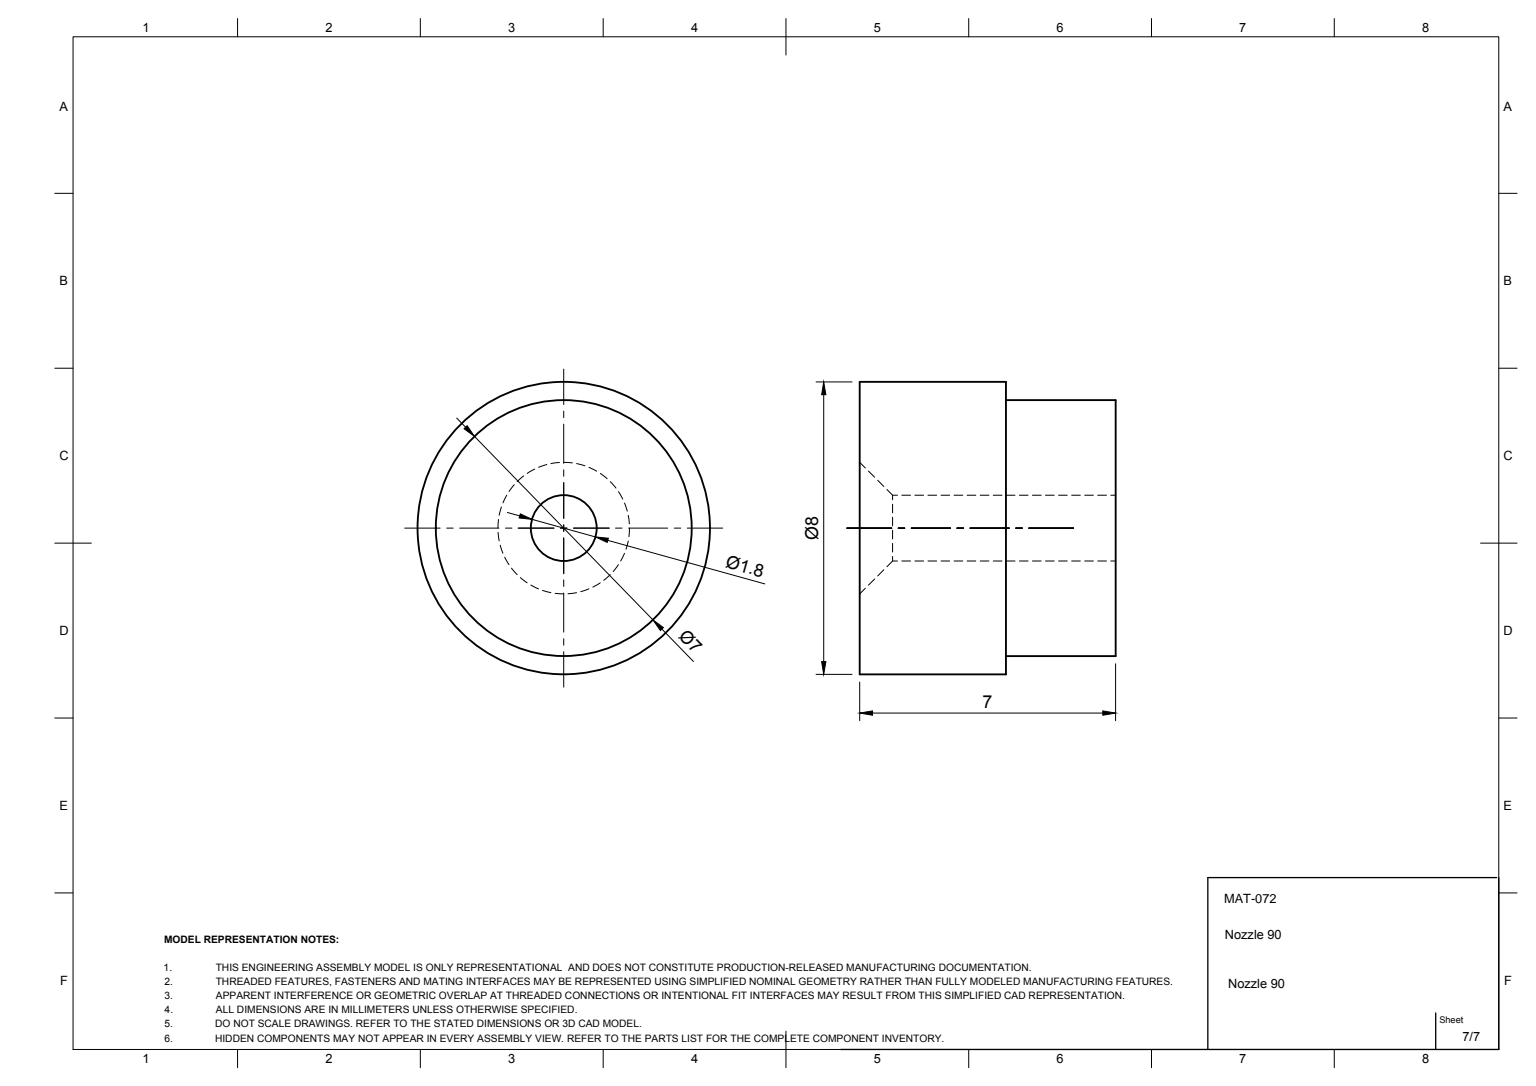
ISO-10303-21;
HEADER;
/* Generated by software containing ST-Developer
 * from STEP Tools, Inc. (www.steptools.com) 
 */

FILE_DESCRIPTION(
/* description */ (''),
/* implementation_level */ '2;1');

FILE_NAME(
/* name */ 'Nozzle 90.step',
/* time_stamp */ '2026-10-24T10:30:45-07:00',
/* author */ (''),
/* organization */ (''),
/* preprocessor_version */ 'ST-DEVELOPER v20.2',
/* originating_system */ 'Autodesk Translation Framework v15.15.0.0',
/* authorisation */ '');

FILE_SCHEMA (('AUTOMOTIVE_DESIGN { 1 0 10303 214 3 1 1 }'));
ENDSEC;

DATA;
#10=MECHANICAL_DESIGN_GEOMETRIC_PRESENTATION_REPRESENTATION('',(#81),#5183);
#66=CONICAL_SURFACE('',#2661,1.8,0.785398163397448);
#71=SHAPE_REPRESENTATION_RELATIONSHIP('SRR','None',#5218,#76);
#76=ADVANCED_BREP_SHAPE_REPRESENTATION('',(#86),#5182);
#81=STYLED_ITEM('',(#5247),#86);
#86=MANIFOLD_SOLID_BREP('Nozzle 90',#2367);
#141=FACE_BOUND('',#598,.T.);
#142=FACE_BOUND('',#600,.T.);
#143=FACE_BOUND('',#604,.T.);
#203=PLANE('',#2654);
#204=PLANE('',#2656);
#205=PLANE('',#2662);
#405=FACE_OUTER_BOUND('',#596,.T.);
#406=FACE_OUTER_BOUND('',#597,.T.);
#407=FACE_OUTER_BOUND('',#599,.T.);
#408=FACE_OUTER_BOUND('',#601,.T.);
#409=FACE_OUTER_BOUND('',#602,.T.);
#410=FACE_OUTER_BOUND('',#603,.T.);
#411=FACE_OUTER_BOUND('',#605,.T.);
#596=EDGE_LOOP('',(#2130,#2131,#2132,#2133));
#597=EDGE_LOOP('',(#2134));
#598=EDGE_LOOP('',(#2135));
#599=EDGE_LOOP('',(#2136));
#600=EDGE_LOOP('',(#2137));
#601=EDGE_LOOP('',(#2138,#2139,#2140,#2141));
#602=EDGE_LOOP('',(#2142,#2143,#2144,#2145));
#603=EDGE_LOOP('',(#2146));
#604=EDGE_LOOP('',(#2147));
#605=EDGE_LOOP('',(#2148,#2149,#2150,#2151));
#697=CIRCLE('',#2652,4.00000000000013);
#698=CIRCLE('',#2653,4.00000000000013);
#699=CIRCLE('',#2655,3.50000000000012);
#700=CIRCLE('',#2657,1.8);
#701=CIRCLE('',#2659,0.89999999999999);
#702=CIRCLE('',#2660,0.899999999999984);
#703=CIRCLE('',#2663,3.50000000000012);
#850=LINE('',#5136,#1000);
#851=LINE('',#5148,#1001);
#852=LINE('',#5151,#1002);
#853=LINE('',#5156,#1003);
#1000=VECTOR('',#3282,4.00000000000013);
#1001=VECTOR('',#3297,0.899999999999984);
#1002=VECTOR('',#3302,1.8);
#1003=VECTOR('',#3309,3.50000000000012);
#1203=VERTEX_POINT('',#5133);
#1204=VERTEX_POINT('',#5135);
#1205=VERTEX_POINT('',#5139);
#1206=VERTEX_POINT('',#5142);
#1207=VERTEX_POINT('',#5145);
#1208=VERTEX_POINT('',#5147);
#1209=VERTEX_POINT('',#5153);
#1513=EDGE_CURVE('',#1203,#1203,#697,.T.);
#1514=EDGE_CURVE('',#1203,#1204,#850,.T.);
#1515=EDGE_CURVE('',#1204,#1204,#698,.T.);
#1516=EDGE_CURVE('',#1205,#1205,#699,.T.);
#1517=EDGE_CURVE('',#1206,#1206,#700,.T.);
#1518=EDGE_CURVE('',#1207,#1207,#701,.T.);
#1519=EDGE_CURVE('',#1207,#1208,#851,.T.);
#1520=EDGE_CURVE('',#1208,#1208,#702,.T.);
#1521=EDGE_CURVE('',#1208,#1206,#852,.T.);
#1522=EDGE_CURVE('',#1209,#1209,#703,.T.);
#1523=EDGE_CURVE('',#1205,#1209,#853,.T.);
#2130=ORIENTED_EDGE('',*,*,#1513,.F.);
#2131=ORIENTED_EDGE('',*,*,#1514,.T.);
#2132=ORIENTED_EDGE('',*,*,#1515,.T.);
#2133=ORIENTED_EDGE('',*,*,#1514,.F.);
#2134=ORIENTED_EDGE('',*,*,#1515,.F.);
#2135=ORIENTED_EDGE('',*,*,#1516,.F.);
#2136=ORIENTED_EDGE('',*,*,#1513,.T.);
#2137=ORIENTED_EDGE('',*,*,#1517,.F.);
#2138=ORIENTED_EDGE('',*,*,#1518,.F.);
#2139=ORIENTED_EDGE('',*,*,#1519,.T.);
#2140=ORIENTED_EDGE('',*,*,#1520,.T.);
#2141=ORIENTED_EDGE('',*,*,#1519,.F.);
#2142=ORIENTED_EDGE('',*,*,#1520,.F.);
#2143=ORIENTED_EDGE('',*,*,#1521,.T.);
#2144=ORIENTED_EDGE('',*,*,#1517,.T.);
#2145=ORIENTED_EDGE('',*,*,#1521,.F.);
#2146=ORIENTED_EDGE('',*,*,#1522,.T.);
#2147=ORIENTED_EDGE('',*,*,#1518,.T.);
#2148=ORIENTED_EDGE('',*,*,#1516,.T.);
#2149=ORIENTED_EDGE('',*,*,#1523,.T.);
#2150=ORIENTED_EDGE('',*,*,#1522,.F.);
#2151=ORIENTED_EDGE('',*,*,#1523,.F.);
#2220=CYLINDRICAL_SURFACE('',#2651,4.00000000000013);
#2221=CYLINDRICAL_SURFACE('',#2658,0.899999999999984);
#2222=CYLINDRICAL_SURFACE('',#2664,3.50000000000012);
#2356=ADVANCED_FACE('',(#405),#2220,.T.);
#2357=ADVANCED_FACE('',(#406,#141),#203,.F.);
#2358=ADVANCED_FACE('',(#407,#142),#204,.T.);
#2359=ADVANCED_FACE('',(#408),#2221,.F.);
#2360=ADVANCED_FACE('',(#409),#66,.F.);
#2361=ADVANCED_FACE('',(#410,#143),#205,.T.);
#2362=ADVANCED_FACE('',(#411),#2222,.T.);
#2367=CLOSED_SHELL('',(#2356,#2357,#2358,#2359,#2360,#2361,#2362));
#2650=AXIS2_PLACEMENT_3D('',#5131,#3276,#3277);
#2651=AXIS2_PLACEMENT_3D('',#5132,#3278,#3279);
#2652=AXIS2_PLACEMENT_3D('',#5134,#3280,#3281);
#2653=AXIS2_PLACEMENT_3D('',#5137,#3283,#3284);
#2654=AXIS2_PLACEMENT_3D('',#5138,#3285,#3286);
#2655=AXIS2_PLACEMENT_3D('',#5140,#3287,#3288);
#2656=AXIS2_PLACEMENT_3D('',#5141,#3289,#3290);
#2657=AXIS2_PLACEMENT_3D('',#5143,#3291,#3292);
#2658=AXIS2_PLACEMENT_3D('',#5144,#3293,#3294);
#2659=AXIS2_PLACEMENT_3D('',#5146,#3295,#3296);
#2660=AXIS2_PLACEMENT_3D('',#5149,#3298,#3299);
#2661=AXIS2_PLACEMENT_3D('',#5150,#3300,#3301);
#2662=AXIS2_PLACEMENT_3D('',#5152,#3303,#3304);
#2663=AXIS2_PLACEMENT_3D('',#5154,#3305,#3306);
#2664=AXIS2_PLACEMENT_3D('',#5155,#3307,#3308);
#3276=DIRECTION('axis',(0.,0.,1.));
#3277=DIRECTION('refdir',(1.,0.,0.));
#3278=DIRECTION('center_axis',(0.,1.,0.));
#3279=DIRECTION('ref_axis',(0.,0.,1.));
#3280=DIRECTION('center_axis',(0.,1.,0.));
#3281=DIRECTION('ref_axis',(0.,0.,1.));
#3282=DIRECTION('',(0.,-1.,0.));
#3283=DIRECTION('center_axis',(0.,1.,0.));
#3284=DIRECTION('ref_axis',(0.,0.,1.));
#3285=DIRECTION('center_axis',(0.,1.,0.));
#3286=DIRECTION('ref_axis',(0.,0.,1.));
#3287=DIRECTION('center_axis',(0.,-1.,0.));
#3288=DIRECTION('ref_axis',(0.,0.,-1.));
#3289=DIRECTION('center_axis',(0.,1.,0.));
#3290=DIRECTION('ref_axis',(0.,0.,1.));
#3291=DIRECTION('center_axis',(0.,1.,0.));
#3292=DIRECTION('ref_axis',(0.,0.,1.));
#3293=DIRECTION('center_axis',(0.,1.,0.));
#3294=DIRECTION('ref_axis',(0.,0.,1.));
#3295=DIRECTION('center_axis',(0.,1.,0.));
#3296=DIRECTION('ref_axis',(0.,0.,1.));
#3297=DIRECTION('',(0.,1.,0.));
#3298=DIRECTION('center_axis',(0.,1.,0.));
#3299=DIRECTION('ref_axis',(0.,0.,1.));
#3300=DIRECTION('center_axis',(0.,1.,0.));
#3301=DIRECTION('ref_axis',(0.,0.,1.));
#3302=DIRECTION('',(-8.65956056235494E-17,0.707106781186548,-0.707106781186548));
#3303=DIRECTION('center_axis',(0.,-1.,0.));
#3304=DIRECTION('ref_axis',(0.,0.,-1.));
#3305=DIRECTION('center_axis',(0.,-1.,0.));
#3306=DIRECTION('ref_axis',(0.,0.,-1.));
#3307=DIRECTION('center_axis',(0.,1.,0.));
#3308=DIRECTION('ref_axis',(0.,0.,1.));
#3309=DIRECTION('',(0.,-1.,0.));
#5131=CARTESIAN_POINT('',(0.,0.,0.));
#5132=CARTESIAN_POINT('Origin',(-75.5607164801933,132.,-55.624999999998));
#5133=CARTESIAN_POINT('',(-75.5607164801933,136.,-59.6249999999981));
#5134=CARTESIAN_POINT('Origin',(-75.5607164801933,136.,-55.624999999998));
#5135=CARTESIAN_POINT('',(-75.5607164801933,132.,-59.6249999999981));
#5136=CARTESIAN_POINT('',(-75.5607164801933,132.,-59.6249999999981));
#5137=CARTESIAN_POINT('Origin',(-75.5607164801933,132.,-55.624999999998));
#5138=CARTESIAN_POINT('Origin',(-75.5607164801933,132.,-55.624999999998));
#5139=CARTESIAN_POINT('',(-75.5607164801933,132.,-59.1249999999981));
#5140=CARTESIAN_POINT('Origin',(-75.5607164801933,132.,-55.624999999998));
#5141=CARTESIAN_POINT('Origin',(-75.5607164801933,136.,-55.624999999998));
#5142=CARTESIAN_POINT('',(-75.5607164801933,136.,-57.424999999998));
#5143=CARTESIAN_POINT('Origin',(-75.5607164801933,136.,-55.624999999998));
#5144=CARTESIAN_POINT('Origin',(-75.5607164801933,136.,-55.624999999998));
#5145=CARTESIAN_POINT('',(-75.5607164801933,129.,-56.524999999998));
#5146=CARTESIAN_POINT('Origin',(-75.5607164801933,129.,-55.624999999998));
#5147=CARTESIAN_POINT('',(-75.5607164801933,135.1,-56.524999999998));
#5148=CARTESIAN_POINT('',(-75.5607164801933,136.,-56.524999999998));
#5149=CARTESIAN_POINT('Origin',(-75.5607164801933,135.1,-55.624999999998));
#5150=CARTESIAN_POINT('Origin',(-75.5607164801933,136.,-55.624999999998));
#5151=CARTESIAN_POINT('',(-75.5607164801933,136.,-57.424999999998));
#5152=CARTESIAN_POINT('Origin',(-75.5607164801933,129.,-55.624999999998));
#5153=CARTESIAN_POINT('',(-75.5607164801933,129.,-59.1249999999981));
#5154=CARTESIAN_POINT('Origin',(-75.5607164801933,129.,-55.624999999998));
#5155=CARTESIAN_POINT('Origin',(-75.5607164801933,129.,-55.624999999998));
#5156=CARTESIAN_POINT('',(-75.5607164801933,129.,-59.1249999999981));
#5175=UNCERTAINTY_MEASURE_WITH_UNIT(LENGTH_MEASURE(0.01),#5184,
'DISTANCE_ACCURACY_VALUE',
'Maximum model space distance between geometric entities at asserted c
onnectivities');
#5176=UNCERTAINTY_MEASURE_WITH_UNIT(LENGTH_MEASURE(0.01),#5184,
'DISTANCE_ACCURACY_VALUE',
'Maximum model space distance between geometric entities at asserted c
onnectivities');
#5182=(
GEOMETRIC_REPRESENTATION_CONTEXT(3)
GLOBAL_UNCERTAINTY_ASSIGNED_CONTEXT((#5175))
GLOBAL_UNIT_ASSIGNED_CONTEXT((#5184,#5186,#5187))
REPRESENTATION_CONTEXT('','3D')
);
#5183=(
GEOMETRIC_REPRESENTATION_CONTEXT(3)
GLOBAL_UNCERTAINTY_ASSIGNED_CONTEXT((#5176))
GLOBAL_UNIT_ASSIGNED_CONTEXT((#5184,#5186,#5187))
REPRESENTATION_CONTEXT('','3D')
);
#5184=(
LENGTH_UNIT()
NAMED_UNIT(*)
SI_UNIT(.MILLI.,.METRE.)
);
#5186=(
NAMED_UNIT(*)
PLANE_ANGLE_UNIT()
SI_UNIT($,.RADIAN.)
);
#5187=(
NAMED_UNIT(*)
SI_UNIT($,.STERADIAN.)
SOLID_ANGLE_UNIT()
);
#5193=SHAPE_DEFINITION_REPRESENTATION(#5199,#5218);
#5199=PRODUCT_DEFINITION_SHAPE('',$,#5225);
#5218=SHAPE_REPRESENTATION('',(#2650),#5182);
#5219=PRODUCT_DEFINITION_CONTEXT('part definition',#5239,'design');
#5225=PRODUCT_DEFINITION('Nozzle 90','Nozzle 90',#5231,#5219);
#5231=PRODUCT_DEFINITION_FORMATION('',$,#5246);
#5239=APPLICATION_CONTEXT(
'Core Data for Automotive Mechanical Design Process');
#5240=PRODUCT_CONTEXT('part definition',#5239,'mechanical');
#5246=PRODUCT('Nozzle 90','Nozzle 90',$,(#5240));
#5247=PRESENTATION_STYLE_ASSIGNMENT((#5248));
#5248=SURFACE_STYLE_USAGE(.BOTH.,#5249);
#5249=SURFACE_SIDE_STYLE('',(#5250));
#5250=SURFACE_STYLE_FILL_AREA(#5251);
#5251=FILL_AREA_STYLE('Steel - Satin',(#5252));
#5252=FILL_AREA_STYLE_COLOUR('Steel - Satin',#5253);
#5253=COLOUR_RGB('Steel - Satin',0.627450980392157,0.627450980392157,0.627450980392157);
ENDSEC;
END-ISO-10303-21;
